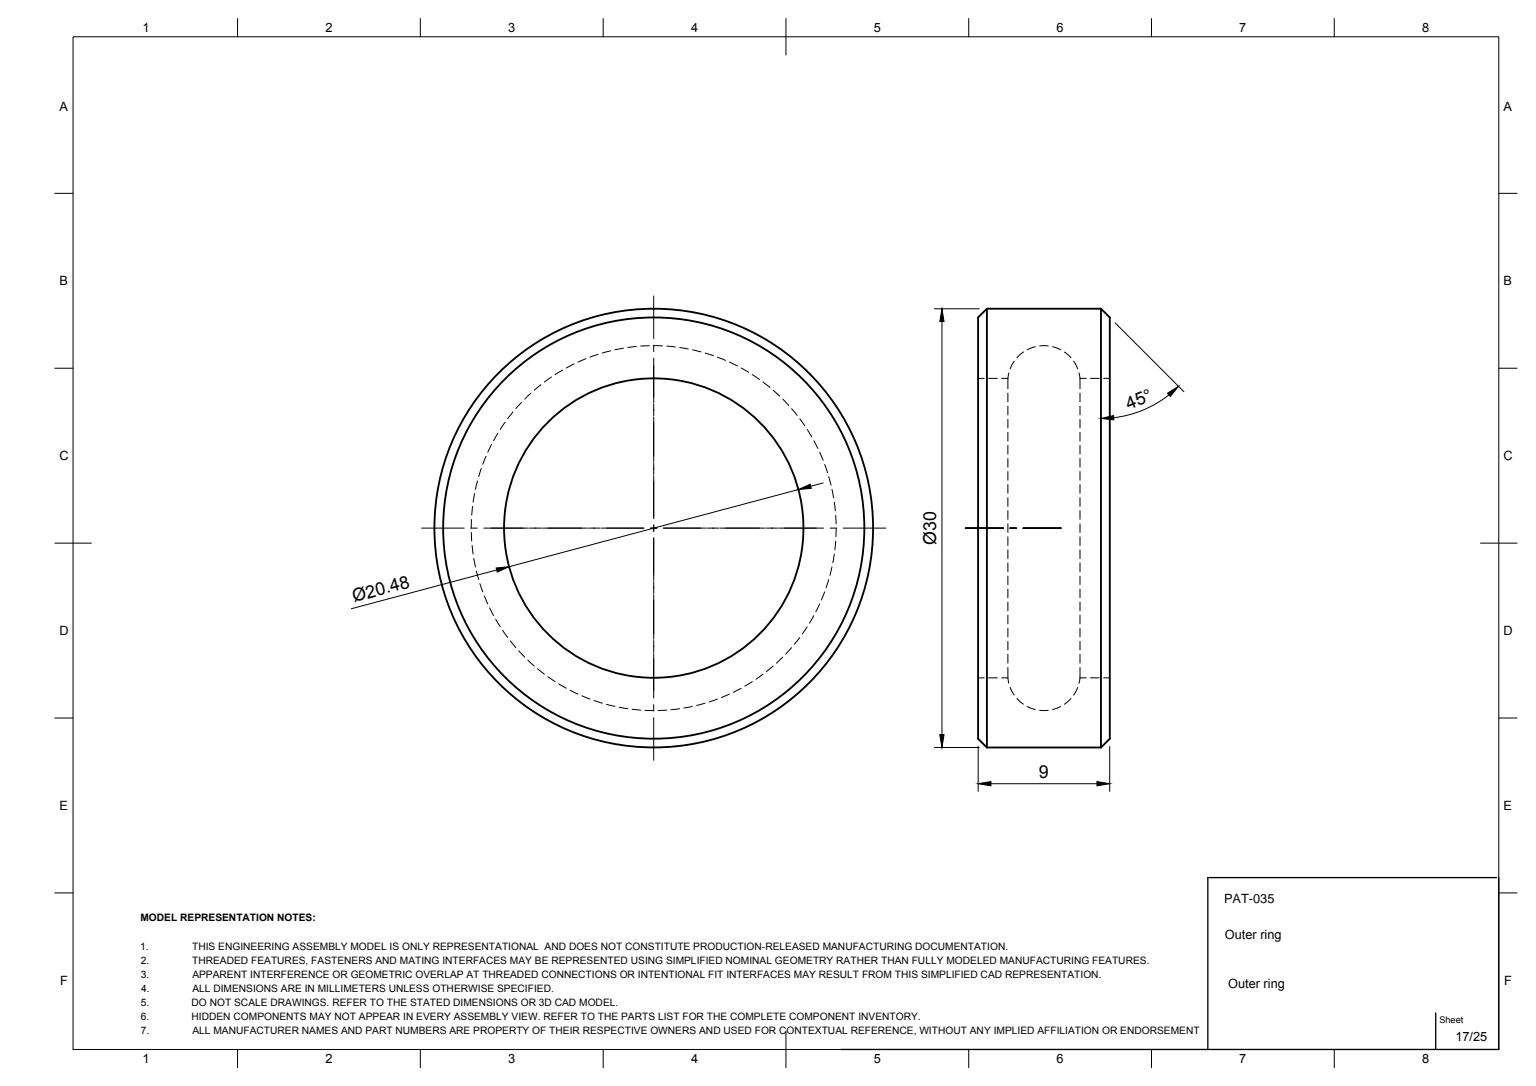
ISO-10303-21;
HEADER;
/* Generated by software containing ST-Developer
 * from STEP Tools, Inc. (www.steptools.com) 
 */

FILE_DESCRIPTION(
/* description */ ('Five-roller gravity conveyor'),
/* implementation_level */ '2;1');

FILE_NAME(
/* name */ 'Outer ring.step',
/* time_stamp */ '2026-10-29T15:36:43-07:00',
/* author */ (''),
/* organization */ (''),
/* preprocessor_version */ 'ST-DEVELOPER v20.2',
/* originating_system */ 'Autodesk Translation Framework v15.17.0.0',
/* authorisation */ '');

FILE_SCHEMA (('AUTOMOTIVE_DESIGN { 1 0 10303 214 3 1 1 }'));
ENDSEC;

DATA;
#10=MECHANICAL_DESIGN_GEOMETRIC_PRESENTATION_REPRESENTATION('',(#319),#7806);
#258=TOROIDAL_SURFACE('',#4640,1.,0.247676);
#266=CONICAL_SURFACE('',#4651,1.47,0.785398163397449);
#267=CONICAL_SURFACE('',#4655,1.47,0.785398163397449);
#283=SHAPE_REPRESENTATION_RELATIONSHIP('SRR','None',#7921,#301);
#301=ADVANCED_BREP_SHAPE_REPRESENTATION('',(#344),#7794);
#319=STYLED_ITEM('',(#8091),#344);
#344=MANIFOLD_SOLID_BREP('Body1',#4207);
#384=FACE_BOUND('',#1047,.T.);
#385=FACE_BOUND('',#1052,.T.);
#483=CIRCLE('',#4641,1.023815);
#484=CIRCLE('',#4642,1.023815);
#485=CIRCLE('',#4643,0.247676);
#486=CIRCLE('',#4644,1.023815);
#487=CIRCLE('',#4645,1.023815);
#488=CIRCLE('',#4647,1.023815);
#489=CIRCLE('',#4649,1.44);
#490=CIRCLE('',#4650,1.023815);
#491=CIRCLE('',#4652,1.5);
#492=CIRCLE('',#4654,1.5);
#493=CIRCLE('',#4656,1.44);
#620=CYLINDRICAL_SURFACE('',#4646,1.023815);
#621=CYLINDRICAL_SURFACE('',#4653,1.5);
#622=CYLINDRICAL_SURFACE('',#4658,1.023815);
#790=FACE_OUTER_BOUND('',#1044,.T.);
#791=FACE_OUTER_BOUND('',#1045,.T.);
#792=FACE_OUTER_BOUND('',#1046,.T.);
#793=FACE_OUTER_BOUND('',#1048,.T.);
#794=FACE_OUTER_BOUND('',#1049,.T.);
#795=FACE_OUTER_BOUND('',#1050,.T.);
#796=FACE_OUTER_BOUND('',#1051,.T.);
#797=FACE_OUTER_BOUND('',#1053,.T.);
#1044=EDGE_LOOP('',(#3452,#3453,#3454,#3455,#3456,#3457));
#1045=EDGE_LOOP('',(#3458,#3459,#3460,#3461,#3462));
#1046=EDGE_LOOP('',(#3463));
#1047=EDGE_LOOP('',(#3464));
#1048=EDGE_LOOP('',(#3465,#3466,#3467,#3468));
#1049=EDGE_LOOP('',(#3469,#3470,#3471,#3472));
#1050=EDGE_LOOP('',(#3473,#3474,#3475,#3476));
#1051=EDGE_LOOP('',(#3477));
#1052=EDGE_LOOP('',(#3478));
#1053=EDGE_LOOP('',(#3479,#3480,#3481,#3482,#3483));
#1460=LINE('',#6959,#1801);
#1461=LINE('',#6968,#1802);
#1462=LINE('',#6972,#1803);
#1463=LINE('',#6976,#1804);
#1464=LINE('',#6979,#1805);
#1801=VECTOR('',#5638,1.023815);
#1802=VECTOR('',#5649,1.47);
#1803=VECTOR('',#5654,1.5);
#1804=VECTOR('',#5659,1.47);
#1805=VECTOR('',#5664,1.023815);
#2088=VERTEX_POINT('',#6947);
#2089=VERTEX_POINT('',#6948);
#2090=VERTEX_POINT('',#6951);
#2091=VERTEX_POINT('',#6953);
#2092=VERTEX_POINT('',#6957);
#2093=VERTEX_POINT('',#6961);
#2094=VERTEX_POINT('',#6963);
#2095=VERTEX_POINT('',#6966);
#2096=VERTEX_POINT('',#6970);
#2097=VERTEX_POINT('',#6974);
#2569=EDGE_CURVE('',#2088,#2089,#483,.T.);
#2570=EDGE_CURVE('',#2089,#2088,#484,.T.);
#2571=EDGE_CURVE('',#2089,#2090,#485,.T.);
#2572=EDGE_CURVE('',#2091,#2090,#486,.T.);
#2573=EDGE_CURVE('',#2090,#2091,#487,.T.);
#2574=EDGE_CURVE('',#2092,#2092,#488,.T.);
#2575=EDGE_CURVE('',#2092,#2091,#1460,.T.);
#2576=EDGE_CURVE('',#2093,#2093,#489,.T.);
#2577=EDGE_CURVE('',#2094,#2094,#490,.T.);
#2578=EDGE_CURVE('',#2095,#2095,#491,.T.);
#2579=EDGE_CURVE('',#2095,#2093,#1461,.T.);
#2580=EDGE_CURVE('',#2096,#2096,#492,.T.);
#2581=EDGE_CURVE('',#2096,#2095,#1462,.T.);
#2582=EDGE_CURVE('',#2097,#2097,#493,.T.);
#2583=EDGE_CURVE('',#2097,#2096,#1463,.T.);
#2584=EDGE_CURVE('',#2088,#2094,#1464,.T.);
#3452=ORIENTED_EDGE('',*,*,#2569,.F.);
#3453=ORIENTED_EDGE('',*,*,#2570,.F.);
#3454=ORIENTED_EDGE('',*,*,#2571,.T.);
#3455=ORIENTED_EDGE('',*,*,#2572,.F.);
#3456=ORIENTED_EDGE('',*,*,#2573,.F.);
#3457=ORIENTED_EDGE('',*,*,#2571,.F.);
#3458=ORIENTED_EDGE('',*,*,#2574,.T.);
#3459=ORIENTED_EDGE('',*,*,#2575,.T.);
#3460=ORIENTED_EDGE('',*,*,#2572,.T.);
#3461=ORIENTED_EDGE('',*,*,#2573,.T.);
#3462=ORIENTED_EDGE('',*,*,#2575,.F.);
#3463=ORIENTED_EDGE('',*,*,#2576,.F.);
#3464=ORIENTED_EDGE('',*,*,#2577,.T.);
#3465=ORIENTED_EDGE('',*,*,#2578,.F.);
#3466=ORIENTED_EDGE('',*,*,#2579,.T.);
#3467=ORIENTED_EDGE('',*,*,#2576,.T.);
#3468=ORIENTED_EDGE('',*,*,#2579,.F.);
#3469=ORIENTED_EDGE('',*,*,#2580,.F.);
#3470=ORIENTED_EDGE('',*,*,#2581,.T.);
#3471=ORIENTED_EDGE('',*,*,#2578,.T.);
#3472=ORIENTED_EDGE('',*,*,#2581,.F.);
#3473=ORIENTED_EDGE('',*,*,#2582,.F.);
#3474=ORIENTED_EDGE('',*,*,#2583,.T.);
#3475=ORIENTED_EDGE('',*,*,#2580,.T.);
#3476=ORIENTED_EDGE('',*,*,#2583,.F.);
#3477=ORIENTED_EDGE('',*,*,#2582,.T.);
#3478=ORIENTED_EDGE('',*,*,#2574,.F.);
#3479=ORIENTED_EDGE('',*,*,#2569,.T.);
#3480=ORIENTED_EDGE('',*,*,#2570,.T.);
#3481=ORIENTED_EDGE('',*,*,#2584,.T.);
#3482=ORIENTED_EDGE('',*,*,#2577,.F.);
#3483=ORIENTED_EDGE('',*,*,#2584,.F.);
#3928=PLANE('',#4648);
#3929=PLANE('',#4657);
#4105=ADVANCED_FACE('',(#790),#258,.F.);
#4106=ADVANCED_FACE('',(#791),#620,.F.);
#4107=ADVANCED_FACE('',(#792,#384),#3928,.T.);
#4108=ADVANCED_FACE('',(#793),#266,.T.);
#4109=ADVANCED_FACE('',(#794),#621,.T.);
#4110=ADVANCED_FACE('',(#795),#267,.T.);
#4111=ADVANCED_FACE('',(#796,#385),#3929,.T.);
#4112=ADVANCED_FACE('',(#797),#622,.F.);
#4207=CLOSED_SHELL('',(#4105,#4106,#4107,#4108,#4109,#4110,#4111,#4112));
#4639=AXIS2_PLACEMENT_3D('',#6945,#5620,#5621);
#4640=AXIS2_PLACEMENT_3D('',#6946,#5622,#5623);
#4641=AXIS2_PLACEMENT_3D('',#6949,#5624,#5625);
#4642=AXIS2_PLACEMENT_3D('',#6950,#5626,#5627);
#4643=AXIS2_PLACEMENT_3D('',#6952,#5628,#5629);
#4644=AXIS2_PLACEMENT_3D('',#6954,#5630,#5631);
#4645=AXIS2_PLACEMENT_3D('',#6955,#5632,#5633);
#4646=AXIS2_PLACEMENT_3D('',#6956,#5634,#5635);
#4647=AXIS2_PLACEMENT_3D('',#6958,#5636,#5637);
#4648=AXIS2_PLACEMENT_3D('',#6960,#5639,#5640);
#4649=AXIS2_PLACEMENT_3D('',#6962,#5641,#5642);
#4650=AXIS2_PLACEMENT_3D('',#6964,#5643,#5644);
#4651=AXIS2_PLACEMENT_3D('',#6965,#5645,#5646);
#4652=AXIS2_PLACEMENT_3D('',#6967,#5647,#5648);
#4653=AXIS2_PLACEMENT_3D('',#6969,#5650,#5651);
#4654=AXIS2_PLACEMENT_3D('',#6971,#5652,#5653);
#4655=AXIS2_PLACEMENT_3D('',#6973,#5655,#5656);
#4656=AXIS2_PLACEMENT_3D('',#6975,#5657,#5658);
#4657=AXIS2_PLACEMENT_3D('',#6977,#5660,#5661);
#4658=AXIS2_PLACEMENT_3D('',#6978,#5662,#5663);
#5620=DIRECTION('axis',(0.,0.,1.));
#5621=DIRECTION('refdir',(1.,0.,0.));
#5622=DIRECTION('center_axis',(0.,-1.,0.));
#5623=DIRECTION('ref_axis',(0.,0.,-1.));
#5624=DIRECTION('center_axis',(0.,-1.,0.));
#5625=DIRECTION('ref_axis',(1.,0.,0.));
#5626=DIRECTION('center_axis',(0.,-1.,0.));
#5627=DIRECTION('ref_axis',(1.,0.,0.));
#5628=DIRECTION('center_axis',(1.,0.,1.22464679914735E-16));
#5629=DIRECTION('ref_axis',(-1.22464679914735E-16,0.,1.));
#5630=DIRECTION('center_axis',(0.,1.,0.));
#5631=DIRECTION('ref_axis',(1.,0.,0.));
#5632=DIRECTION('center_axis',(0.,1.,0.));
#5633=DIRECTION('ref_axis',(1.,0.,0.));
#5634=DIRECTION('center_axis',(0.,-1.,0.));
#5635=DIRECTION('ref_axis',(1.,0.,0.));
#5636=DIRECTION('center_axis',(0.,-1.,0.));
#5637=DIRECTION('ref_axis',(1.,0.,0.));
#5638=DIRECTION('',(0.,1.,0.));
#5639=DIRECTION('center_axis',(0.,1.,0.));
#5640=DIRECTION('ref_axis',(0.,0.,1.));
#5641=DIRECTION('center_axis',(0.,-1.,0.));
#5642=DIRECTION('ref_axis',(1.,0.,0.));
#5643=DIRECTION('center_axis',(0.,-1.,0.));
#5644=DIRECTION('ref_axis',(1.,0.,0.));
#5645=DIRECTION('center_axis',(0.,-1.,0.));
#5646=DIRECTION('ref_axis',(1.,0.,0.));
#5647=DIRECTION('center_axis',(0.,-1.,0.));
#5648=DIRECTION('ref_axis',(1.,0.,0.));
#5649=DIRECTION('',(0.707106781186548,0.707106781186547,8.65956056235494E-17));
#5650=DIRECTION('center_axis',(0.,-1.,0.));
#5651=DIRECTION('ref_axis',(1.,0.,0.));
#5652=DIRECTION('center_axis',(0.,-1.,0.));
#5653=DIRECTION('ref_axis',(1.,0.,0.));
#5654=DIRECTION('',(0.,1.,0.));
#5655=DIRECTION('center_axis',(0.,1.,0.));
#5656=DIRECTION('ref_axis',(1.,0.,0.));
#5657=DIRECTION('center_axis',(0.,-1.,0.));
#5658=DIRECTION('ref_axis',(1.,0.,0.));
#5659=DIRECTION('',(-0.707106781186548,0.707106781186547,-8.65956056235494E-17));
#5660=DIRECTION('center_axis',(0.,-1.,0.));
#5661=DIRECTION('ref_axis',(0.,0.,-1.));
#5662=DIRECTION('center_axis',(0.,-1.,0.));
#5663=DIRECTION('ref_axis',(1.,0.,0.));
#5664=DIRECTION('',(0.,1.,0.));
#6945=CARTESIAN_POINT('',(0.,0.,0.));
#6946=CARTESIAN_POINT('Origin',(0.,0.,0.));
#6947=CARTESIAN_POINT('',(-1.023815,0.246528389340863,-1.25381176266905E-16));
#6948=CARTESIAN_POINT('',(-1.25381176266905E-16,0.246528389340863,1.023815));
#6949=CARTESIAN_POINT('Origin',(0.,0.246528389340863,0.));
#6950=CARTESIAN_POINT('Origin',(0.,0.246528389340863,0.));
#6951=CARTESIAN_POINT('',(-1.25381176266905E-16,-0.246528389340863,1.023815));
#6952=CARTESIAN_POINT('Origin',(-1.22464679914735E-16,0.,1.));
#6953=CARTESIAN_POINT('',(-1.023815,-0.246528389340863,1.25381176266905E-16));
#6954=CARTESIAN_POINT('Origin',(0.,-0.246528389340863,0.));
#6955=CARTESIAN_POINT('Origin',(0.,-0.246528389340863,0.));
#6956=CARTESIAN_POINT('Origin',(0.,0.,0.));
#6957=CARTESIAN_POINT('',(-1.023815,-0.45,-1.25381176266905E-16));
#6958=CARTESIAN_POINT('Origin',(0.,-0.45,0.));
#6959=CARTESIAN_POINT('',(-1.023815,0.,-1.25381176266905E-16));
#6960=CARTESIAN_POINT('Origin',(1.44,0.45,0.));
#6961=CARTESIAN_POINT('',(-1.44,0.45,-1.76349139077219E-16));
#6962=CARTESIAN_POINT('Origin',(0.,0.45,0.));
#6963=CARTESIAN_POINT('',(-1.023815,0.45,-1.25381176266905E-16));
#6964=CARTESIAN_POINT('Origin',(0.,0.45,0.));
#6965=CARTESIAN_POINT('Origin',(0.,0.42,0.));
#6966=CARTESIAN_POINT('',(-1.5,0.39,-1.83697019872103E-16));
#6967=CARTESIAN_POINT('Origin',(0.,0.39,0.));
#6968=CARTESIAN_POINT('',(-1.47,0.42,-1.80023079474661E-16));
#6969=CARTESIAN_POINT('Origin',(0.,0.,0.));
#6970=CARTESIAN_POINT('',(-1.5,-0.39,-1.83697019872103E-16));
#6971=CARTESIAN_POINT('Origin',(0.,-0.39,0.));
#6972=CARTESIAN_POINT('',(-1.5,0.,-1.83697019872103E-16));
#6973=CARTESIAN_POINT('Origin',(0.,-0.42,0.));
#6974=CARTESIAN_POINT('',(-1.44,-0.45,-1.76349139077219E-16));
#6975=CARTESIAN_POINT('Origin',(0.,-0.45,0.));
#6976=CARTESIAN_POINT('',(-1.47,-0.42,-1.80023079474661E-16));
#6977=CARTESIAN_POINT('Origin',(1.023815,-0.45,0.));
#6978=CARTESIAN_POINT('Origin',(0.,0.,0.));
#6979=CARTESIAN_POINT('',(-1.023815,0.,-1.25381176266905E-16));
#7770=UNCERTAINTY_MEASURE_WITH_UNIT(LENGTH_MEASURE(0.001),#7807,
'DISTANCE_ACCURACY_VALUE',
'Maximum model space distance between geometric entities at asserted c
onnectivities');
#7782=UNCERTAINTY_MEASURE_WITH_UNIT(LENGTH_MEASURE(0.001),#7807,
'DISTANCE_ACCURACY_VALUE',
'Maximum model space distance between geometric entities at asserted c
onnectivities');
#7794=(
GEOMETRIC_REPRESENTATION_CONTEXT(3)
GLOBAL_UNCERTAINTY_ASSIGNED_CONTEXT((#7770))
GLOBAL_UNIT_ASSIGNED_CONTEXT((#7807,#7809,#7810))
REPRESENTATION_CONTEXT('','3D')
);
#7806=(
GEOMETRIC_REPRESENTATION_CONTEXT(3)
GLOBAL_UNCERTAINTY_ASSIGNED_CONTEXT((#7782))
GLOBAL_UNIT_ASSIGNED_CONTEXT((#7807,#7809,#7810))
REPRESENTATION_CONTEXT('','3D')
);
#7807=(
LENGTH_UNIT()
NAMED_UNIT(*)
SI_UNIT(.CENTI.,.METRE.)
);
#7809=(
NAMED_UNIT(*)
PLANE_ANGLE_UNIT()
SI_UNIT($,.RADIAN.)
);
#7810=(
NAMED_UNIT(*)
SI_UNIT($,.STERADIAN.)
SOLID_ANGLE_UNIT()
);
#7822=SHAPE_DEFINITION_REPRESENTATION(#7845,#7921);
#7845=PRODUCT_DEFINITION_SHAPE('',$,#7945);
#7921=SHAPE_REPRESENTATION('',(#4639),#7794);
#7933=PRODUCT_DEFINITION_CONTEXT('part definition',#8004,'design');
#7945=PRODUCT_DEFINITION('Outer ring','Outer ring',#7968,#7933);
#7968=PRODUCT_DEFINITION_FORMATION('',$,#8017);
#8004=APPLICATION_CONTEXT(
'Core Data for Automotive Mechanical Design Process');
#8005=PRODUCT_CONTEXT('part definition',#8004,'mechanical');
#8017=PRODUCT('Outer ring','Outer ring','Outer ring',(#8005));
#8085=COLOUR_RGB('Grey',0.48,0.52,0.57);
#8086=FILL_AREA_STYLE_COLOUR('',#8085);
#8087=FILL_AREA_STYLE('',(#8086));
#8088=SURFACE_STYLE_FILL_AREA(#8087);
#8089=SURFACE_SIDE_STYLE('',(#8088));
#8090=SURFACE_STYLE_USAGE(.BOTH.,#8089);
#8091=PRESENTATION_STYLE_ASSIGNMENT((#8090));
ENDSEC;
END-ISO-10303-21;
